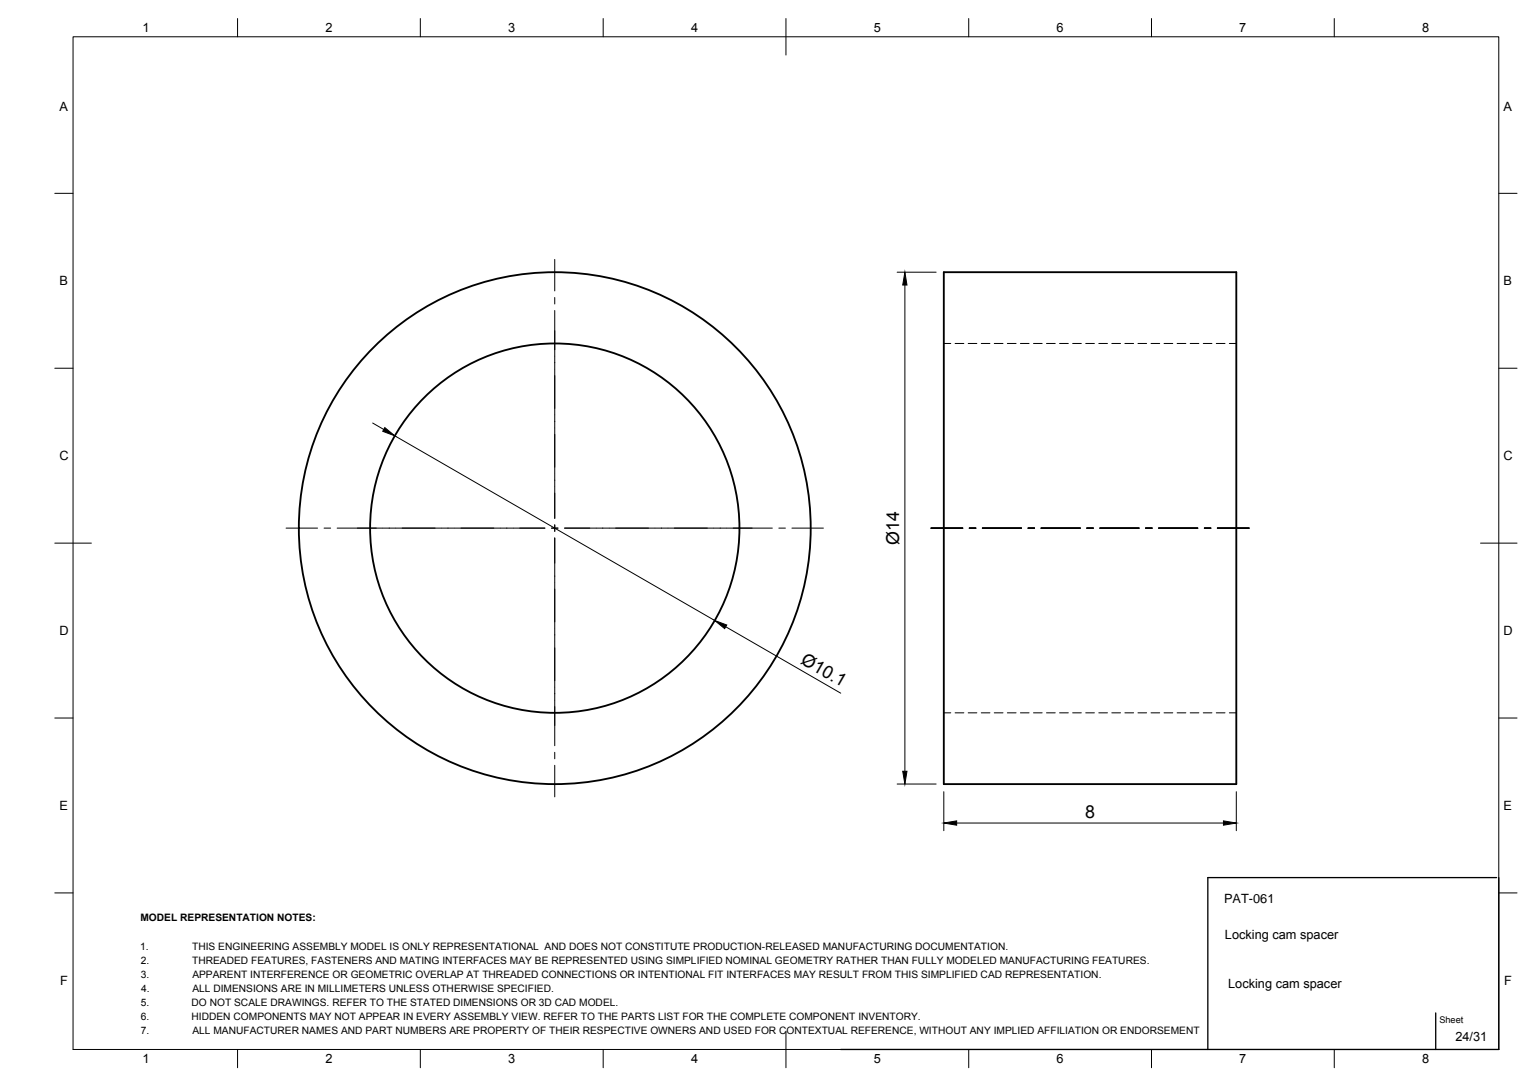
ISO-10303-21;
HEADER;
/* Generated by software containing ST-Developer
 * from STEP Tools, Inc. (www.steptools.com) 
 */

FILE_DESCRIPTION(
/* description */ ('Compact intermittent indexer'),
/* implementation_level */ '2;1');

FILE_NAME(
/* name */ 'Locking cam spacer.step',
/* time_stamp */ '2026-10-29T16:32:17-07:00',
/* author */ (''),
/* organization */ (''),
/* preprocessor_version */ 'ST-DEVELOPER v20.2',
/* originating_system */ 'Autodesk Translation Framework v15.17.0.0',
/* authorisation */ '');

FILE_SCHEMA (('AUTOMOTIVE_DESIGN { 1 0 10303 214 3 1 1 }'));
ENDSEC;

DATA;
#10=MECHANICAL_DESIGN_GEOMETRIC_PRESENTATION_REPRESENTATION('',(#281),#10837);
#225=SHAPE_REPRESENTATION_RELATIONSHIP('SRR','None',#10961,#249);
#249=ADVANCED_BREP_SHAPE_REPRESENTATION('',(#312),#10828);
#281=STYLED_ITEM('',(#11180),#312);
#312=MANIFOLD_SOLID_BREP('Body1',#5654);
#448=FACE_BOUND('',#1302,.T.);
#449=FACE_BOUND('',#1304,.T.);
#583=PLANE('',#6423);
#584=PLANE('',#6424);
#876=FACE_OUTER_BOUND('',#1299,.T.);
#877=FACE_OUTER_BOUND('',#1300,.T.);
#878=FACE_OUTER_BOUND('',#1301,.T.);
#879=FACE_OUTER_BOUND('',#1303,.T.);
#1299=EDGE_LOOP('',(#4636,#4637,#4638,#4639));
#1300=EDGE_LOOP('',(#4640,#4641,#4642,#4643));
#1301=EDGE_LOOP('',(#4644));
#1302=EDGE_LOOP('',(#4645));
#1303=EDGE_LOOP('',(#4646));
#1304=EDGE_LOOP('',(#4647));
#1627=LINE('',#10061,#1985);
#1628=LINE('',#10067,#1986);
#1985=VECTOR('',#7843,0.505);
#1986=VECTOR('',#7850,0.7);
#2387=CIRCLE('',#6418,0.505);
#2388=CIRCLE('',#6419,0.505);
#2389=CIRCLE('',#6421,0.7);
#2390=CIRCLE('',#6422,0.7);
#2799=VERTEX_POINT('',#10058);
#2800=VERTEX_POINT('',#10060);
#2801=VERTEX_POINT('',#10064);
#2802=VERTEX_POINT('',#10066);
#3440=EDGE_CURVE('',#2799,#2799,#2387,.T.);
#3441=EDGE_CURVE('',#2799,#2800,#1627,.T.);
#3442=EDGE_CURVE('',#2800,#2800,#2388,.T.);
#3443=EDGE_CURVE('',#2801,#2801,#2389,.T.);
#3444=EDGE_CURVE('',#2801,#2802,#1628,.T.);
#3445=EDGE_CURVE('',#2802,#2802,#2390,.T.);
#4636=ORIENTED_EDGE('',*,*,#3440,.F.);
#4637=ORIENTED_EDGE('',*,*,#3441,.T.);
#4638=ORIENTED_EDGE('',*,*,#3442,.T.);
#4639=ORIENTED_EDGE('',*,*,#3441,.F.);
#4640=ORIENTED_EDGE('',*,*,#3443,.F.);
#4641=ORIENTED_EDGE('',*,*,#3444,.T.);
#4642=ORIENTED_EDGE('',*,*,#3445,.T.);
#4643=ORIENTED_EDGE('',*,*,#3444,.F.);
#4644=ORIENTED_EDGE('',*,*,#3443,.T.);
#4645=ORIENTED_EDGE('',*,*,#3440,.T.);
#4646=ORIENTED_EDGE('',*,*,#3445,.F.);
#4647=ORIENTED_EDGE('',*,*,#3442,.F.);
#5258=CYLINDRICAL_SURFACE('',#6417,0.505);
#5259=CYLINDRICAL_SURFACE('',#6420,0.7);
#5519=ADVANCED_FACE('',(#876),#5258,.F.);
#5520=ADVANCED_FACE('',(#877),#5259,.T.);
#5521=ADVANCED_FACE('',(#878,#448),#583,.T.);
#5522=ADVANCED_FACE('',(#879,#449),#584,.F.);
#5654=CLOSED_SHELL('',(#5519,#5520,#5521,#5522));
#6416=AXIS2_PLACEMENT_3D('',#10056,#7837,#7838);
#6417=AXIS2_PLACEMENT_3D('',#10057,#7839,#7840);
#6418=AXIS2_PLACEMENT_3D('',#10059,#7841,#7842);
#6419=AXIS2_PLACEMENT_3D('',#10062,#7844,#7845);
#6420=AXIS2_PLACEMENT_3D('',#10063,#7846,#7847);
#6421=AXIS2_PLACEMENT_3D('',#10065,#7848,#7849);
#6422=AXIS2_PLACEMENT_3D('',#10068,#7851,#7852);
#6423=AXIS2_PLACEMENT_3D('',#10069,#7853,#7854);
#6424=AXIS2_PLACEMENT_3D('',#10070,#7855,#7856);
#7837=DIRECTION('axis',(0.,0.,1.));
#7838=DIRECTION('refdir',(1.,0.,0.));
#7839=DIRECTION('center_axis',(0.,0.,1.));
#7840=DIRECTION('ref_axis',(1.,0.,0.));
#7841=DIRECTION('center_axis',(0.,0.,-1.));
#7842=DIRECTION('ref_axis',(1.,0.,0.));
#7843=DIRECTION('',(0.,0.,-1.));
#7844=DIRECTION('center_axis',(0.,0.,-1.));
#7845=DIRECTION('ref_axis',(1.,0.,0.));
#7846=DIRECTION('center_axis',(0.,0.,1.));
#7847=DIRECTION('ref_axis',(1.,0.,0.));
#7848=DIRECTION('center_axis',(0.,0.,1.));
#7849=DIRECTION('ref_axis',(1.,0.,0.));
#7850=DIRECTION('',(0.,0.,-1.));
#7851=DIRECTION('center_axis',(0.,0.,1.));
#7852=DIRECTION('ref_axis',(1.,0.,0.));
#7853=DIRECTION('center_axis',(0.,0.,1.));
#7854=DIRECTION('ref_axis',(1.,0.,0.));
#7855=DIRECTION('center_axis',(0.,0.,1.));
#7856=DIRECTION('ref_axis',(1.,0.,0.));
#10056=CARTESIAN_POINT('',(0.,0.,0.));
#10057=CARTESIAN_POINT('Origin',(0.,0.,5.2));
#10058=CARTESIAN_POINT('',(-0.505,-6.18446633569413E-17,6.));
#10059=CARTESIAN_POINT('Origin',(0.,0.,6.));
#10060=CARTESIAN_POINT('',(-0.505,-6.18446633569413E-17,5.2));
#10061=CARTESIAN_POINT('',(-0.505,-6.18446633569413E-17,5.2));
#10062=CARTESIAN_POINT('Origin',(0.,0.,5.2));
#10063=CARTESIAN_POINT('Origin',(0.,0.,5.2));
#10064=CARTESIAN_POINT('',(-0.7,-8.57252759403147E-17,6.));
#10065=CARTESIAN_POINT('Origin',(0.,0.,6.));
#10066=CARTESIAN_POINT('',(-0.7,-8.57252759403147E-17,5.2));
#10067=CARTESIAN_POINT('',(-0.7,-8.57252759403147E-17,5.2));
#10068=CARTESIAN_POINT('Origin',(0.,0.,5.2));
#10069=CARTESIAN_POINT('Origin',(0.,0.,6.));
#10070=CARTESIAN_POINT('Origin',(0.,0.,5.2));
#10798=UNCERTAINTY_MEASURE_WITH_UNIT(LENGTH_MEASURE(0.001),#10838,
'DISTANCE_ACCURACY_VALUE',
'Maximum model space distance between geometric entities at asserted c
onnectivities');
#10807=UNCERTAINTY_MEASURE_WITH_UNIT(LENGTH_MEASURE(0.001),#10838,
'DISTANCE_ACCURACY_VALUE',
'Maximum model space distance between geometric entities at asserted c
onnectivities');
#10828=(
GEOMETRIC_REPRESENTATION_CONTEXT(3)
GLOBAL_UNCERTAINTY_ASSIGNED_CONTEXT((#10798))
GLOBAL_UNIT_ASSIGNED_CONTEXT((#10838,#10840,#10841))
REPRESENTATION_CONTEXT('','3D')
);
#10837=(
GEOMETRIC_REPRESENTATION_CONTEXT(3)
GLOBAL_UNCERTAINTY_ASSIGNED_CONTEXT((#10807))
GLOBAL_UNIT_ASSIGNED_CONTEXT((#10838,#10840,#10841))
REPRESENTATION_CONTEXT('','3D')
);
#10838=(
LENGTH_UNIT()
NAMED_UNIT(*)
SI_UNIT(.CENTI.,.METRE.)
);
#10840=(
NAMED_UNIT(*)
PLANE_ANGLE_UNIT()
SI_UNIT($,.RADIAN.)
);
#10841=(
NAMED_UNIT(*)
SI_UNIT($,.STERADIAN.)
SOLID_ANGLE_UNIT()
);
#10862=SHAPE_DEFINITION_REPRESENTATION(#10896,#10961);
#10896=PRODUCT_DEFINITION_SHAPE('',$,#10991);
#10961=SHAPE_REPRESENTATION('',(#6416),#10828);
#10970=PRODUCT_DEFINITION_CONTEXT('part definition',#11059,'design');
#10991=PRODUCT_DEFINITION('Locking cam spacer','Locking cam spacer',#11020,
#10970);
#11020=PRODUCT_DEFINITION_FORMATION('',$,#11081);
#11059=APPLICATION_CONTEXT(
'Core Data for Automotive Mechanical Design Process');
#11060=PRODUCT_CONTEXT('part definition',#11059,'mechanical');
#11081=PRODUCT('Locking cam spacer','Locking cam spacer',
'Locking cam spacer',(#11060));
#11174=COLOUR_RGB('Off White',0.89,0.88,0.83);
#11175=FILL_AREA_STYLE_COLOUR('',#11174);
#11176=FILL_AREA_STYLE('',(#11175));
#11177=SURFACE_STYLE_FILL_AREA(#11176);
#11178=SURFACE_SIDE_STYLE('',(#11177));
#11179=SURFACE_STYLE_USAGE(.BOTH.,#11178);
#11180=PRESENTATION_STYLE_ASSIGNMENT((#11179));
ENDSEC;
END-ISO-10303-21;
